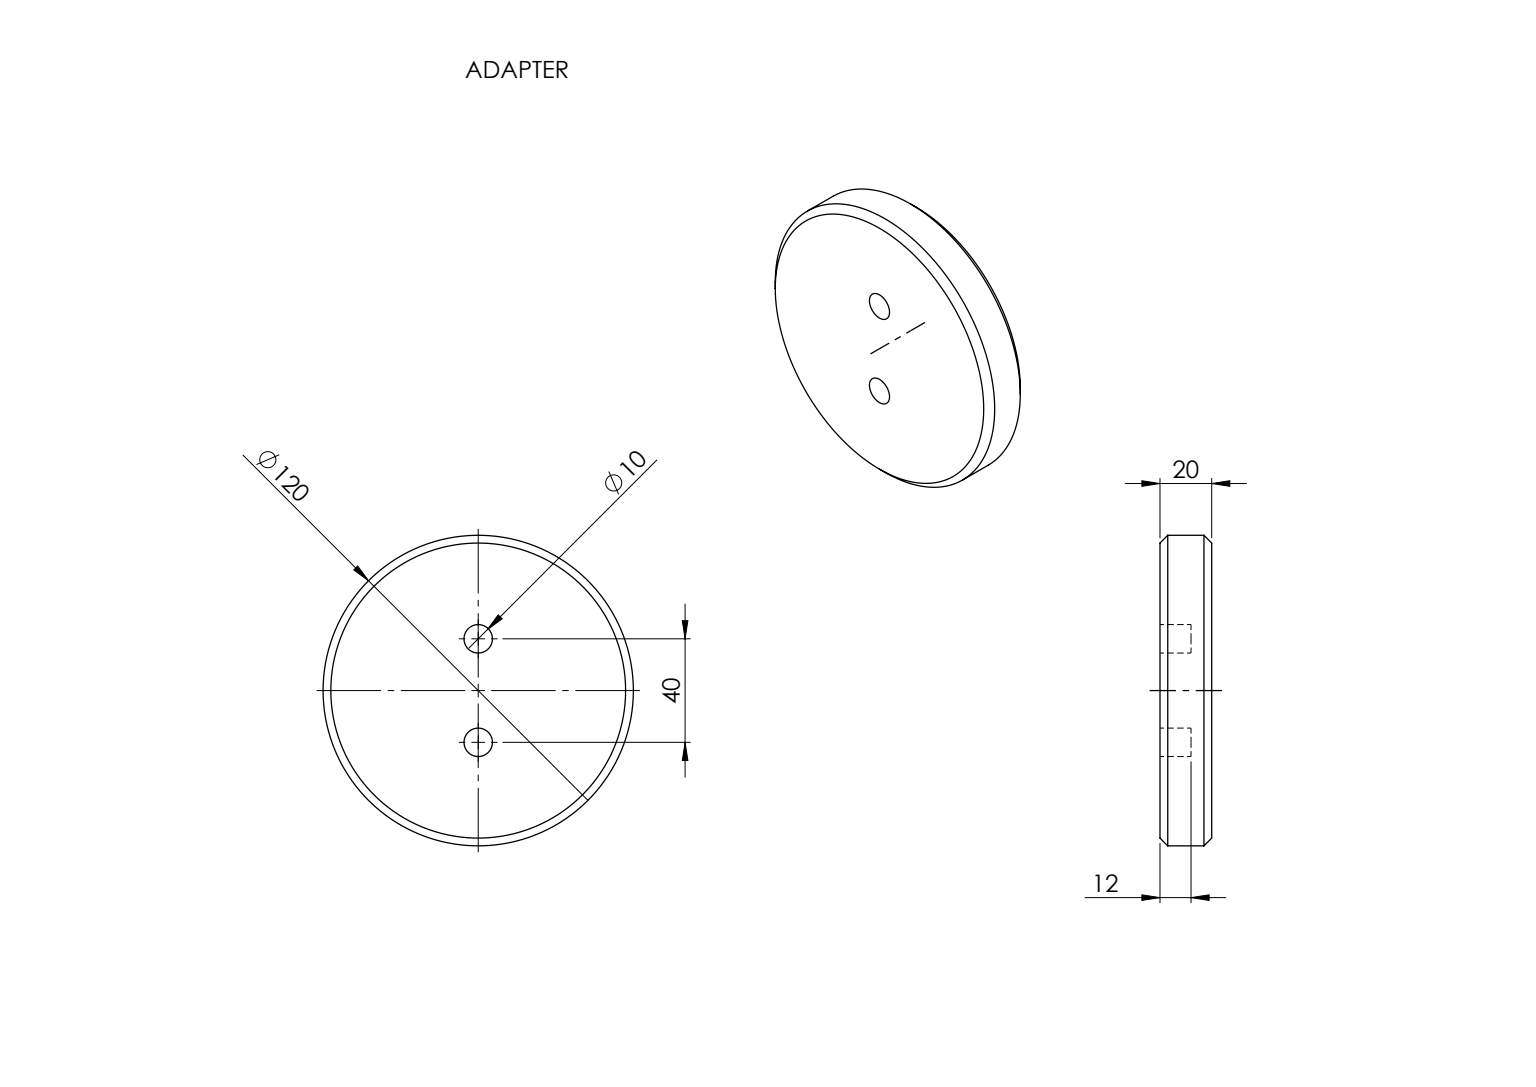
ISO-10303-21;
HEADER;
FILE_DESCRIPTION (('STEP AP203'),
    '1' );
FILE_NAME ('adapter.step',
    '2026-09-28T05:57:06',
    ( '' ),
    ( '' ),
    'SwSTEP 2.0',
    'SolidWorks 2026',
    '' );
FILE_SCHEMA (( 'AUTOMOTIVE_DESIGN' ));
ENDSEC;

DATA;
#193=DIRECTION ( 'NONE',  ( -1.000000000000000000, 0.000000000000000000, 0.000000000000000000 ) ) ;
#236=CARTESIAN_POINT ( 'NONE',  ( 57.00000000000002132, 7.164183775012018789E-15, -220.0000000000000000 ) ) ;
#380=VECTOR ( 'NONE', #39658, 1000.000000000000000 ) ;
#484=ORIENTED_EDGE ( 'NONE', *, *, #2776, .T. ) ;
#740=VERTEX_POINT ( 'NONE', #18224 ) ;
#960=LINE ( 'NONE', #1170, #21072 ) ;
#1101=VECTOR ( 'NONE', #34234, 1000.000000000000114 ) ;
#1161=ORIENTED_EDGE ( 'NONE', *, *, #15645, .F. ) ;
#1170=CARTESIAN_POINT ( 'NONE',  ( -60.00000000000000711, 0.000000000000000000, -223.0000000000000000 ) ) ;
#1309=ORIENTED_EDGE ( 'NONE', *, *, #22453, .T. ) ;
#1322=ORIENTED_EDGE ( 'NONE', *, *, #12215, .F. ) ;
#1370=EDGE_CURVE ( 'NONE', #2118, #27376, #40003, .T. ) ;
#1394=DIRECTION ( 'NONE',  ( -0.000000000000000000, -0.000000000000000000, -1.000000000000000000 ) ) ;
#1563=CIRCLE ( 'NONE', #31918, 57.00000000000002132 ) ;
#1637=VERTEX_POINT ( 'NONE', #18825 ) ;
#1639=CARTESIAN_POINT ( 'NONE',  ( -5.500000000000005329, -20.00000000000000000, -232.0000000000000000 ) ) ;
#1658=APPLICATION_CONTEXT ( 'configuration controlled 3d designs of mechanical parts and assemblies' ) ;
#1713=DIRECTION ( 'NONE',  ( -0.000000000000000000, -0.000000000000000000, -1.000000000000000000 ) ) ;
#1847=CIRCLE ( 'NONE', #5285, 5.500000000000003553 ) ;
#2045=DIRECTION ( 'NONE',  ( -1.000000000000000000, 0.000000000000000000, 0.000000000000000000 ) ) ;
#2118=VERTEX_POINT ( 'NONE', #23558 ) ;
#2181=DIRECTION ( 'NONE',  ( 1.000000000000000000, 0.000000000000000000, 0.000000000000000000 ) ) ;
#2233=CARTESIAN_POINT ( 'NONE',  ( -2.275517850991317657E-15, -20.00000000000000000, -220.0000000000000000 ) ) ;
#2248=CONICAL_SURFACE ( 'NONE', #30493, 57.00000000000002132, 0.7853981633974401744 ) ;
#2458=CARTESIAN_POINT ( 'NONE',  ( -5.500000000000003553, 20.00000000000000000, -220.0000000000000000 ) ) ;
#2487=ORIENTED_EDGE ( 'NONE', *, *, #39307, .F. ) ;
#2493=VERTEX_POINT ( 'NONE', #33169 ) ;
#2732=EDGE_CURVE ( 'NONE', #23382, #12287, #31420, .T. ) ;
#2776=EDGE_CURVE ( 'NONE', #32481, #2118, #24311, .T. ) ;
#2835=DIRECTION ( 'NONE',  ( 0.000000000000000000, 0.000000000000000000, 1.000000000000000000 ) ) ;
#2858=EDGE_CURVE ( 'NONE', #23382, #9326, #21044, .T. ) ;
#3002=ADVANCED_FACE ( 'NONE', ( #15827 ), #29024, .T. ) ;
#3318=CARTESIAN_POINT ( 'NONE',  ( -5.500000000000003553, 20.00000000000000000, -232.0000000000000000 ) ) ;
#3346=CARTESIAN_POINT ( 'NONE',  ( 0.000000000000000000, 20.00000000000000000, -232.0000000000000000 ) ) ;
#3794=PLANE ( 'NONE',  #12718 ) ;
#4148=CARTESIAN_POINT ( 'NONE',  ( 0.000000000000000000, 0.000000000000000000, -220.0000000000000000 ) ) ;
#4242=CONICAL_SURFACE ( 'NONE', #10452, 57.00000000000002132, 0.7853981633974401744 ) ;
#4358=EDGE_CURVE ( 'NONE', #35303, #32901, #36921, .T. ) ;
#4359=DIRECTION ( 'NONE',  ( 0.000000000000000000, 0.000000000000000000, 1.000000000000000000 ) ) ;
#4514=CYLINDRICAL_SURFACE ( 'NONE', #40311, 5.500000000000003553 ) ;
#4553=EDGE_LOOP ( 'NONE', ( #1161, #17163, #11750, #29234 ) ) ;
#5020=DIRECTION ( 'NONE',  ( -0.000000000000000000, -0.000000000000000000, 1.000000000000000000 ) ) ;
#5285=AXIS2_PLACEMENT_3D ( 'NONE', #30798, #38119, #21284 ) ;
#5507=DIRECTION ( 'NONE',  ( 1.000000000000000000, 0.000000000000000000, 0.000000000000000000 ) ) ;
#5518=CONICAL_SURFACE ( 'NONE', #26890, 60.00000000000000711, 0.7853981633974447263 ) ;
#5527=ADVANCED_FACE ( 'NONE', ( #23729 ), #15687, .T. ) ;
#5532=DIRECTION ( 'NONE',  ( 1.000000000000000000, 0.000000000000000000, 0.000000000000000000 ) ) ;
#5685=VERTEX_POINT ( 'NONE', #40743 ) ;
#5789=LINE ( 'NONE', #22397, #7054 ) ;
#6235=DIRECTION ( 'NONE',  ( -0.000000000000000000, -0.000000000000000000, 1.000000000000000000 ) ) ;
#6283=DESIGN_CONTEXT ( 'detailed design', #1658, 'design' ) ;
#6358=AXIS2_PLACEMENT_3D ( 'NONE', #35803, #6235, #193 ) ;
#6631=AXIS2_PLACEMENT_3D ( 'NONE', #37693, #15007, #5532 ) ;
#6876=CIRCLE ( 'NONE', #24103, 5.500000000000003553 ) ;
#6903=CARTESIAN_POINT ( 'NONE',  ( 0.000000000000000000, 0.000000000000000000, -236.9999999999999716 ) ) ;
#7054=VECTOR ( 'NONE', #35785, 1000.000000000000000 ) ;
#7543=FACE_OUTER_BOUND ( 'NONE', #32058, .T. ) ;
#7844=DIRECTION ( 'NONE',  ( -0.000000000000000000, -0.000000000000000000, -1.000000000000000000 ) ) ;
#7898=DIRECTION ( 'NONE',  ( -0.000000000000000000, -0.000000000000000000, 1.000000000000000000 ) ) ;
#8122=DIRECTION ( 'NONE',  ( -0.000000000000000000, -0.000000000000000000, 1.000000000000000000 ) ) ;
#8208=ORIENTED_EDGE ( 'NONE', *, *, #4358, .F. ) ;
#8316=DIRECTION ( 'NONE',  ( 0.000000000000000000, 0.000000000000000000, 1.000000000000000000 ) ) ;
#8492=VERTEX_POINT ( 'NONE', #25338 ) ;
#8866=ORIENTED_EDGE ( 'NONE', *, *, #28211, .T. ) ;
#9072=ORIENTED_EDGE ( 'NONE', *, *, #9834, .F. ) ;
#9326=VERTEX_POINT ( 'NONE', #15542 ) ;
#9491=ORIENTED_EDGE ( 'NONE', *, *, #2858, .T. ) ;
#9834=EDGE_CURVE ( 'NONE', #8492, #5685, #20607, .T. ) ;
#10053=CARTESIAN_POINT ( 'NONE',  ( 60.00000000000000711, 0.000000000000000000, -240.0000000000000000 ) ) ;
#10073=CIRCLE ( 'NONE', #6631, 5.500000000000003553 ) ;
#10213=ORIENTED_EDGE ( 'NONE', *, *, #4358, .T. ) ;
#10322=DIRECTION ( 'NONE',  ( 1.000000000000000000, 0.000000000000000000, 0.000000000000000000 ) ) ;
#10407=ORIENTED_EDGE ( 'NONE', *, *, #16935, .T. ) ;
#10452=AXIS2_PLACEMENT_3D ( 'NONE', #22039, #11663, #35000 ) ;
#10532=ORIENTED_EDGE ( 'NONE', *, *, #33338, .F. ) ;
#10620=EDGE_CURVE ( 'NONE', #5685, #8492, #31701, .T. ) ;
#10627=CARTESIAN_POINT ( 'NONE',  ( 0.000000000000000000, 0.000000000000000000, -223.0000000000000000 ) ) ;
#10691=ORIENTED_EDGE ( 'NONE', *, *, #18172, .T. ) ;
#10913=CYLINDRICAL_SURFACE ( 'NONE', #42182, 5.500000000000003553 ) ;
#10977=DIRECTION ( 'NONE',  ( 1.000000000000000000, 0.000000000000000000, 0.000000000000000000 ) ) ;
#11045=ORIENTED_EDGE ( 'NONE', *, *, #19567, .T. ) ;
#11112=DIRECTION ( 'NONE',  ( 0.000000000000000000, 0.000000000000000000, 1.000000000000000000 ) ) ;
#11162=LINE ( 'NONE', #15034, #36535 ) ;
#11383=ADVANCED_FACE ( 'NONE', ( #21403 ), #24880, .T. ) ;
#11396=DIRECTION ( 'NONE',  ( -1.000000000000000000, 0.000000000000000000, 0.000000000000000000 ) ) ;
#11462=FACE_BOUND ( 'NONE', #29875, .T. ) ;
#11630=ORIENTED_EDGE ( 'NONE', *, *, #12241, .F. ) ;
#11663=DIRECTION ( 'NONE',  ( 0.000000000000000000, 0.000000000000000000, 1.000000000000000000 ) ) ;
#11697=DIRECTION ( 'NONE',  ( 1.000000000000000000, 0.000000000000000000, 0.000000000000000000 ) ) ;
#11750=ORIENTED_EDGE ( 'NONE', *, *, #29145, .T. ) ;
#11756=AXIS2_PLACEMENT_3D ( 'NONE', #2233, #28556, #11697 ) ;
#11785=( GEOMETRIC_REPRESENTATION_CONTEXT ( 3 ) GLOBAL_UNCERTAINTY_ASSIGNED_CONTEXT ( ( #12723 ) ) GLOBAL_UNIT_ASSIGNED_CONTEXT ( ( #35513, #38737, #42168 ) ) REPRESENTATION_CONTEXT ( 'NONE', 'WORKASPACE' ) );
#11914=CARTESIAN_POINT ( 'NONE',  ( -2.275517850991317657E-15, -20.00000000000000000, -232.0000000000000000 ) ) ;
#11964=ORIENTED_EDGE ( 'NONE', *, *, #38901, .F. ) ;
#11965=DIRECTION ( 'NONE',  ( 0.000000000000000000, 0.000000000000000000, -1.000000000000000000 ) ) ;
#12025=DIRECTION ( 'NONE',  ( -0.000000000000000000, -0.000000000000000000, -1.000000000000000000 ) ) ;
#12215=EDGE_CURVE ( 'NONE', #740, #35303, #32992, .T. ) ;
#12241=EDGE_CURVE ( 'NONE', #2493, #27376, #26304, .T. ) ;
#12275=CYLINDRICAL_SURFACE ( 'NONE', #24306, 60.00000000000000711 ) ;
#12287=VERTEX_POINT ( 'NONE', #25670 ) ;
#12718=AXIS2_PLACEMENT_3D ( 'NONE', #21678, #8316, #37442 ) ;
#12723=UNCERTAINTY_MEASURE_WITH_UNIT (LENGTH_MEASURE( 1.000000000000000082E-05 ), #35513, 'distance_accuracy_value', 'NONE');
#12816=SHAPE_REPRESENTATION ( 'adapter', ( #39998 ), #11785 ) ;
#13120=FACE_OUTER_BOUND ( 'NONE', #29690, .T. ) ;
#13284=ADVANCED_FACE ( 'NONE', ( #33374 ), #3794, .T. ) ;
#13467=APPLICATION_CONTEXT ( 'configuration controlled 3d designs of mechanical parts and assemblies' ) ;
#13471=EDGE_LOOP ( 'NONE', ( #17054, #40046, #32542, #32157 ) ) ;
#14188=CARTESIAN_POINT ( 'NONE',  ( 0.000000000000000000, 0.000000000000000000, -223.0000000000000000 ) ) ;
#14397=VERTEX_POINT ( 'NONE', #27211 ) ;
#14563=PRODUCT ( 'adapter', 'adapter', '', ( #16678 ) ) ;
#14656=ORIENTED_EDGE ( 'NONE', *, *, #2732, .F. ) ;
#14767=CARTESIAN_POINT ( 'NONE',  ( 60.00000000000000711, 7.347880794884119933E-15, -223.0000000000000000 ) ) ;
#15007=DIRECTION ( 'NONE',  ( 0.000000000000000000, 0.000000000000000000, 1.000000000000000000 ) ) ;
#15034=CARTESIAN_POINT ( 'NONE',  ( -60.00000000000000711, 7.347880794884119933E-15, -240.0000000000000000 ) ) ;
#15040=CARTESIAN_POINT ( 'NONE',  ( 0.000000000000000000, 0.000000000000000000, -223.0000000000000000 ) ) ;
#15044=AXIS2_PLACEMENT_3D ( 'NONE', #3346, #20365, #23413 ) ;
#15410=CARTESIAN_POINT ( 'NONE',  ( 0.000000000000000000, 0.000000000000000000, -240.0000000000000000 ) ) ;
#15415=SHAPE_REPRESENTATION_RELATIONSHIP ( 'NONE' , 'NONE' ,  #12816, #16028 ) ;
#15542=CARTESIAN_POINT ( 'NONE',  ( 60.00000000000000711, 0.000000000000000000, -223.0000000000000000 ) ) ;
#15645=EDGE_CURVE ( 'NONE', #14397, #5685, #20828, .T. ) ;
#15687=CONICAL_SURFACE ( 'NONE', #28110, 60.00000000000000711, 0.7853981633974447263 ) ;
#15820=DIRECTION ( 'NONE',  ( -0.000000000000000000, -0.000000000000000000, 1.000000000000000000 ) ) ;
#15827=FACE_OUTER_BOUND ( 'NONE', #35717, .T. ) ;
#15849=DIRECTION ( 'NONE',  ( 1.000000000000000000, 0.000000000000000000, -0.000000000000000000 ) ) ;
#15921=PRODUCT_DEFINITION ( 'UNKNOWN', '', #36593, #6283 ) ;
#16028=ADVANCED_BREP_SHAPE_REPRESENTATION ( '', ( #29947, #39998 ), #11785 ) ;
#16120=CARTESIAN_POINT ( 'NONE',  ( -60.00000000000000711, 7.347880794884119933E-15, -223.0000000000000000 ) ) ;
#16275=ADVANCED_FACE ( 'NONE', ( #27640 ), #2248, .T. ) ;
#16443=ORIENTED_EDGE ( 'NONE', *, *, #22506, .F. ) ;
#16678=MECHANICAL_CONTEXT ( 'NONE', #13467, 'mechanical' ) ;
#16734=VERTEX_POINT ( 'NONE', #16120 ) ;
#16893=AXIS2_PLACEMENT_3D ( 'NONE', #25601, #26229, #15849 ) ;
#16935=EDGE_CURVE ( 'NONE', #12287, #23382, #24986, .T. ) ;
#17054=ORIENTED_EDGE ( 'NONE', *, *, #41015, .F. ) ;
#17100=CIRCLE ( 'NONE', #41223, 5.500000000000003553 ) ;
#17163=ORIENTED_EDGE ( 'NONE', *, *, #18172, .F. ) ;
#17263=AXIS2_PLACEMENT_3D ( 'NONE', #39888, #26527, #10322 ) ;
#17268=ORIENTED_EDGE ( 'NONE', *, *, #39307, .T. ) ;
#17292=DIRECTION ( 'NONE',  ( 0.000000000000000000, 0.000000000000000000, -1.000000000000000000 ) ) ;
#17389=AXIS2_PLACEMENT_3D ( 'NONE', #22480, #35023, #35656 ) ;
#17585=AXIS2_PLACEMENT_3D ( 'NONE', #28290, #31537, #2181 ) ;
#18033=CIRCLE ( 'NONE', #29768, 5.500000000000003553 ) ;
#18147=EDGE_CURVE ( 'NONE', #14397, #1637, #1563, .T. ) ;
#18172=EDGE_CURVE ( 'NONE', #1637, #14397, #25684, .T. ) ;
#18224=CARTESIAN_POINT ( 'NONE',  ( 5.500000000000003553, 20.00000000000000000, -232.0000000000000000 ) ) ;
#18549=DIRECTION ( 'NONE',  ( 1.000000000000000000, 0.000000000000000000, 0.000000000000000000 ) ) ;
#18619=ADVANCED_FACE ( 'NONE', ( #41630 ), #12275, .T. ) ;
#18825=CARTESIAN_POINT ( 'NONE',  ( 57.00000000000002132, 0.000000000000000000, -240.0000000000000000 ) ) ;
#19040=ORIENTED_EDGE ( 'NONE', *, *, #41015, .T. ) ;
#19111=PLANE ( 'NONE',  #16893 ) ;
#19567=EDGE_CURVE ( 'NONE', #12287, #16734, #960, .T. ) ;
#19669=ORIENTED_EDGE ( 'NONE', *, *, #25456, .T. ) ;
#19683=VECTOR ( 'NONE', #7898, 1000.000000000000000 ) ;
#20127=ORIENTED_EDGE ( 'NONE', *, *, #18147, .F. ) ;
#20365=DIRECTION ( 'NONE',  ( -0.000000000000000000, -0.000000000000000000, 1.000000000000000000 ) ) ;
#20607=CIRCLE ( 'NONE', #34440, 60.00000000000000711 ) ;
#20828=LINE ( 'NONE', #31208, #36662 ) ;
#20970=FACE_OUTER_BOUND ( 'NONE', #27807, .T. ) ;
#21016=CARTESIAN_POINT ( 'NONE',  ( 0.000000000000000000, 0.000000000000000000, -223.0000000000000000 ) ) ;
#21044=LINE ( 'NONE', #14767, #1101 ) ;
#21072=VECTOR ( 'NONE', #24049, 1000.000000000000114 ) ;
#21276=AXIS2_PLACEMENT_3D ( 'NONE', #29585, #2835, #25721 ) ;
#21284=DIRECTION ( 'NONE',  ( 1.000000000000000000, 0.000000000000000000, 0.000000000000000000 ) ) ;
#21318=EDGE_LOOP ( 'NONE', ( #8208, #41075 ) ) ;
#21403=FACE_OUTER_BOUND ( 'NONE', #13471, .T. ) ;
#21493=CARTESIAN_POINT ( 'NONE',  ( 0.000000000000000000, 20.00000000000000000, -232.0000000000000000 ) ) ;
#21678=CARTESIAN_POINT ( 'NONE',  ( 0.000000000000000000, 20.00000000000000000, -232.0000000000000000 ) ) ;
#21837=DIRECTION ( 'NONE',  ( 1.000000000000000000, 0.000000000000000000, 0.000000000000000000 ) ) ;
#21844=CARTESIAN_POINT ( 'NONE',  ( 0.000000000000000000, 0.000000000000000000, -240.0000000000000000 ) ) ;
#21902=DIRECTION ( 'NONE',  ( 0.000000000000000000, 0.000000000000000000, 1.000000000000000000 ) ) ;
#22039=CARTESIAN_POINT ( 'NONE',  ( 0.000000000000000000, 0.000000000000000000, -240.0000000000000000 ) ) ;
#22127=ORIENTED_EDGE ( 'NONE', *, *, #29145, .F. ) ;
#22183=EDGE_LOOP ( 'NONE', ( #16443, #19669, #8866, #1322 ) ) ;
#22220=CARTESIAN_POINT ( 'NONE',  ( 0.000000000000000000, 0.000000000000000000, -240.0000000000000000 ) ) ;
#22268=CARTESIAN_POINT ( 'NONE',  ( 0.000000000000000000, 0.000000000000000000, -240.0000000000000000 ) ) ;
#22397=CARTESIAN_POINT ( 'NONE',  ( 57.00000000000002132, 0.000000000000000000, -240.0000000000000000 ) ) ;
#22444=EDGE_LOOP ( 'NONE', ( #17268, #41777 ) ) ;
#22453=EDGE_CURVE ( 'NONE', #740, #40819, #10073, .T. ) ;
#22480=CARTESIAN_POINT ( 'NONE',  ( 0.000000000000000000, 0.000000000000000000, -240.0000000000000000 ) ) ;
#22506=EDGE_CURVE ( 'NONE', #40819, #740, #1847, .T. ) ;
#22812=ADVANCED_FACE ( 'NONE', ( #29253 ), #19111, .T. ) ;
#23024=CARTESIAN_POINT ( 'NONE',  ( 0.000000000000000000, 0.000000000000000000, -220.0000000000000000 ) ) ;
#23134=ORIENTED_EDGE ( 'NONE', *, *, #19567, .F. ) ;
#23272=DIRECTION ( 'NONE',  ( -0.000000000000000000, -0.000000000000000000, 1.000000000000000000 ) ) ;
#23382=VERTEX_POINT ( 'NONE', #236 ) ;
#23413=DIRECTION ( 'NONE',  ( 1.000000000000000000, 0.000000000000000000, 0.000000000000000000 ) ) ;
#23558=CARTESIAN_POINT ( 'NONE',  ( -5.500000000000005329, -20.00000000000000000, -220.0000000000000000 ) ) ;
#23563=ORIENTED_EDGE ( 'NONE', *, *, #15645, .T. ) ;
#23591=ADVANCED_FACE ( 'NONE', ( #7543 ), #4514, .F. ) ;
#23644=ORIENTED_EDGE ( 'NONE', *, *, #22453, .F. ) ;
#23729=FACE_OUTER_BOUND ( 'NONE', #36978, .T. ) ;
#23792=FACE_BOUND ( 'NONE', #21318, .T. ) ;
#23829=AXIS2_PLACEMENT_3D ( 'NONE', #23024, #29715, #39831 ) ;
#24049=DIRECTION ( 'NONE',  ( -0.7071067811865451302, 0.000000000000000000, -0.7071067811865500152 ) ) ;
#24103=AXIS2_PLACEMENT_3D ( 'NONE', #11914, #38255, #28773 ) ;
#24229=PLANE ( 'NONE',  #25009 ) ;
#24306=AXIS2_PLACEMENT_3D ( 'NONE', #22220, #31950, #18549 ) ;
#24311=LINE ( 'NONE', #1639, #19683 ) ;
#24322=DIRECTION ( 'NONE',  ( 1.000000000000000000, 0.000000000000000000, 0.000000000000000000 ) ) ;
#24421=CARTESIAN_POINT ( 'NONE',  ( 0.000000000000000000, 0.000000000000000000, -240.0000000000000000 ) ) ;
#24577=DIRECTION ( 'NONE',  ( -1.000000000000000000, 0.000000000000000000, 0.000000000000000000 ) ) ;
#24743=CARTESIAN_POINT ( 'NONE',  ( 0.000000000000000000, 0.000000000000000000, 0.000000000000000000 ) ) ;
#24846=DIRECTION ( 'NONE',  ( 1.000000000000000000, 0.000000000000000000, 0.000000000000000000 ) ) ;
#24880=CYLINDRICAL_SURFACE ( 'NONE', #36889, 60.00000000000000711 ) ;
#24960=PRODUCT_DEFINITION_SHAPE ( 'NONE', 'NONE',  #15921 ) ;
#24986=CIRCLE ( 'NONE', #6358, 57.00000000000002132 ) ;
#25009=AXIS2_PLACEMENT_3D ( 'NONE', #4148, #17292, #27029 ) ;
#25194=EDGE_LOOP ( 'NONE', ( #20127, #23563, #9072, #22127 ) ) ;
#25338=CARTESIAN_POINT ( 'NONE',  ( 60.00000000000000711, 0.000000000000000000, -236.9999999999999716 ) ) ;
#25456=EDGE_CURVE ( 'NONE', #40819, #32901, #42363, .T. ) ;
#25601=CARTESIAN_POINT ( 'NONE',  ( -2.275517850991317657E-15, -20.00000000000000000, -232.0000000000000000 ) ) ;
#25670=CARTESIAN_POINT ( 'NONE',  ( -57.00000000000002132, 0.000000000000000000, -220.0000000000000000 ) ) ;
#25684=CIRCLE ( 'NONE', #17389, 57.00000000000002132 ) ;
#25721=DIRECTION ( 'NONE',  ( 1.000000000000000000, 0.000000000000000000, 0.000000000000000000 ) ) ;
#25731=DIRECTION ( 'NONE',  ( -1.000000000000000000, 0.000000000000000000, 0.000000000000000000 ) ) ;
#25846=ORIENTED_EDGE ( 'NONE', *, *, #1370, .F. ) ;
#25849=VECTOR ( 'NONE', #23272, 1000.000000000000000 ) ;
#26229=DIRECTION ( 'NONE',  ( 0.000000000000000000, 0.000000000000000000, 1.000000000000000000 ) ) ;
#26304=LINE ( 'NONE', #42049, #380 ) ;
#26467=LINE ( 'NONE', #10053, #38727 ) ;
#26527=DIRECTION ( 'NONE',  ( -0.000000000000000000, -0.000000000000000000, 1.000000000000000000 ) ) ;
#26775=ADVANCED_FACE ( 'NONE', ( #28738 ), #4242, .T. ) ;
#26857=AXIS2_PLACEMENT_3D ( 'NONE', #10627, #7844, #27905 ) ;
#26890=AXIS2_PLACEMENT_3D ( 'NONE', #15040, #12025, #24577 ) ;
#26945=ORIENTED_EDGE ( 'NONE', *, *, #27596, .F. ) ;
#26963=DIRECTION ( 'NONE',  ( 0.000000000000000000, 0.000000000000000000, 1.000000000000000000 ) ) ;
#27029=DIRECTION ( 'NONE',  ( -1.000000000000000000, 0.000000000000000000, -0.000000000000000000 ) ) ;
#27059=SHAPE_DEFINITION_REPRESENTATION ( #24960, #12816 ) ;
#27118=FACE_OUTER_BOUND ( 'NONE', #35922, .T. ) ;
#27211=CARTESIAN_POINT ( 'NONE',  ( -57.00000000000002132, 7.164183775012018789E-15, -240.0000000000000000 ) ) ;
#27274=AXIS2_PLACEMENT_3D ( 'NONE', #15410, #11965, #42163 ) ;
#27376=VERTEX_POINT ( 'NONE', #38150 ) ;
#27478=CIRCLE ( 'NONE', #21276, 5.500000000000003553 ) ;
#27596=EDGE_CURVE ( 'NONE', #8492, #9326, #26467, .T. ) ;
#27640=FACE_OUTER_BOUND ( 'NONE', #25194, .T. ) ;
#27750=ORIENTED_EDGE ( 'NONE', *, *, #1370, .T. ) ;
#27805=FACE_OUTER_BOUND ( 'NONE', #31001, .T. ) ;
#27807=EDGE_LOOP ( 'NONE', ( #10407, #32438 ) ) ;
#27905=DIRECTION ( 'NONE',  ( -1.000000000000000000, 0.000000000000000000, 0.000000000000000000 ) ) ;
#28070=CLOSED_SHELL ( 'NONE', ( #32298, #23591, #16275, #39638, #18619, #11383, #3002, #28357, #5527, #26775, #41929, #22812, #29648, #13284 ) ) ;
#28110=AXIS2_PLACEMENT_3D ( 'NONE', #14188, #1713, #11396 ) ;
#28131=ORIENTED_EDGE ( 'NONE', *, *, #12241, .T. ) ;
#28211=EDGE_CURVE ( 'NONE', #32901, #35303, #18033, .T. ) ;
#28287=DIRECTION ( 'NONE',  ( 0.000000000000000000, 0.000000000000000000, 1.000000000000000000 ) ) ;
#28290=CARTESIAN_POINT ( 'NONE',  ( 0.000000000000000000, 20.00000000000000000, -220.0000000000000000 ) ) ;
#28357=ADVANCED_FACE ( 'NONE', ( #23792, #11462, #20970 ), #24229, .F. ) ;
#28372=DIRECTION ( 'NONE',  ( 0.000000000000000000, 0.000000000000000000, 1.000000000000000000 ) ) ;
#28556=DIRECTION ( 'NONE',  ( 0.000000000000000000, 0.000000000000000000, 1.000000000000000000 ) ) ;
#28738=FACE_OUTER_BOUND ( 'NONE', #4553, .T. ) ;
#28773=DIRECTION ( 'NONE',  ( 1.000000000000000000, 0.000000000000000000, 0.000000000000000000 ) ) ;
#29024=PLANE ( 'NONE',  #27274 ) ;
#29145=EDGE_CURVE ( 'NONE', #1637, #8492, #5789, .T. ) ;
#29234=ORIENTED_EDGE ( 'NONE', *, *, #10620, .F. ) ;
#29253=FACE_OUTER_BOUND ( 'NONE', #22444, .T. ) ;
#29585=CARTESIAN_POINT ( 'NONE',  ( -2.275517850991317657E-15, -20.00000000000000000, -220.0000000000000000 ) ) ;
#29648=ADVANCED_FACE ( 'NONE', ( #27118 ), #10913, .F. ) ;
#29690=EDGE_LOOP ( 'NONE', ( #40460, #2487, #28131, #31427 ) ) ;
#29715=DIRECTION ( 'NONE',  ( -0.000000000000000000, -0.000000000000000000, 1.000000000000000000 ) ) ;
#29768=AXIS2_PLACEMENT_3D ( 'NONE', #41737, #21902, #5507 ) ;
#29875=EDGE_LOOP ( 'NONE', ( #34877, #25846 ) ) ;
#29947=MANIFOLD_SOLID_BREP ( 'Cut-Extrude1', #28070 ) ;
#30493=AXIS2_PLACEMENT_3D ( 'NONE', #24421, #28287, #24846 ) ;
#30666=ORIENTED_EDGE ( 'NONE', *, *, #25456, .F. ) ;
#30776=DIRECTION ( 'NONE',  ( -0.7071067811865417996, 8.659560562354863833E-17, 0.7071067811865532349 ) ) ;
#30798=CARTESIAN_POINT ( 'NONE',  ( 0.000000000000000000, 20.00000000000000000, -232.0000000000000000 ) ) ;
#31001=EDGE_LOOP ( 'NONE', ( #14656, #9491, #42149, #23134 ) ) ;
#31125=VECTOR ( 'NONE', #15820, 1000.000000000000000 ) ;
#31208=CARTESIAN_POINT ( 'NONE',  ( -57.00000000000002132, 6.980486755139916067E-15, -240.0000000000000000 ) ) ;
#31420=CIRCLE ( 'NONE', #23829, 57.00000000000002132 ) ;
#31427=ORIENTED_EDGE ( 'NONE', *, *, #34897, .T. ) ;
#31537=DIRECTION ( 'NONE',  ( 0.000000000000000000, 0.000000000000000000, 1.000000000000000000 ) ) ;
#31701=CIRCLE ( 'NONE', #39255, 60.00000000000000711 ) ;
#31918=AXIS2_PLACEMENT_3D ( 'NONE', #21844, #38672, #25731 ) ;
#31950=DIRECTION ( 'NONE',  ( -0.000000000000000000, -0.000000000000000000, 1.000000000000000000 ) ) ;
#32058=EDGE_LOOP ( 'NONE', ( #10532, #484, #27750, #11630 ) ) ;
#32157=ORIENTED_EDGE ( 'NONE', *, *, #38901, .T. ) ;
#32298=ADVANCED_FACE ( 'NONE', ( #40008 ), #36355, .F. ) ;
#32438=ORIENTED_EDGE ( 'NONE', *, *, #2732, .T. ) ;
#32481=VERTEX_POINT ( 'NONE', #40214 ) ;
#32542=ORIENTED_EDGE ( 'NONE', *, *, #27596, .T. ) ;
#32790=CYLINDRICAL_SURFACE ( 'NONE', #17263, 5.500000000000003553 ) ;
#32901=VERTEX_POINT ( 'NONE', #2458 ) ;
#32992=LINE ( 'NONE', #42468, #25849 ) ;
#33169=CARTESIAN_POINT ( 'NONE',  ( 5.500000000000000888, -20.00000000000000000, -232.0000000000000000 ) ) ;
#33232=ORIENTED_EDGE ( 'NONE', *, *, #12215, .T. ) ;
#33338=EDGE_CURVE ( 'NONE', #32481, #2493, #17100, .T. ) ;
#33374=FACE_OUTER_BOUND ( 'NONE', #40398, .T. ) ;
#33463=CARTESIAN_POINT ( 'NONE',  ( -2.275517850991317657E-15, -20.00000000000000000, -232.0000000000000000 ) ) ;
#33874=EDGE_CURVE ( 'NONE', #16734, #9326, #39208, .T. ) ;
#33935=CARTESIAN_POINT ( 'NONE',  ( -2.275517850991317657E-15, -20.00000000000000000, -232.0000000000000000 ) ) ;
#34234=DIRECTION ( 'NONE',  ( 0.7071067811865451302, 8.659560562354904508E-17, -0.7071067811865500152 ) ) ;
#34319=CARTESIAN_POINT ( 'NONE',  ( 5.500000000000003553, 20.00000000000000000, -220.0000000000000000 ) ) ;
#34440=AXIS2_PLACEMENT_3D ( 'NONE', #6903, #26963, #36679 ) ;
#34877=ORIENTED_EDGE ( 'NONE', *, *, #34897, .F. ) ;
#34897=EDGE_CURVE ( 'NONE', #27376, #2118, #27478, .T. ) ;
#35000=DIRECTION ( 'NONE',  ( 1.000000000000000000, 0.000000000000000000, 0.000000000000000000 ) ) ;
#35023=DIRECTION ( 'NONE',  ( 0.000000000000000000, 0.000000000000000000, -1.000000000000000000 ) ) ;
#35303=VERTEX_POINT ( 'NONE', #34319 ) ;
#35488=CARTESIAN_POINT ( 'NONE',  ( 0.000000000000000000, 0.000000000000000000, -236.9999999999999716 ) ) ;
#35513=( LENGTH_UNIT ( ) NAMED_UNIT ( * ) SI_UNIT ( .MILLI., .METRE. ) );
#35656=DIRECTION ( 'NONE',  ( -1.000000000000000000, 0.000000000000000000, 0.000000000000000000 ) ) ;
#35717=EDGE_LOOP ( 'NONE', ( #10691, #38745 ) ) ;
#35785=DIRECTION ( 'NONE',  ( 0.7071067811865417996, 0.000000000000000000, 0.7071067811865532349 ) ) ;
#35803=CARTESIAN_POINT ( 'NONE',  ( 0.000000000000000000, 0.000000000000000000, -220.0000000000000000 ) ) ;
#35922=EDGE_LOOP ( 'NONE', ( #30666, #23644, #33232, #10213 ) ) ;
#36156=ORIENTED_EDGE ( 'NONE', *, *, #22506, .T. ) ;
#36355=CYLINDRICAL_SURFACE ( 'NONE', #15044, 5.500000000000003553 ) ;
#36535=VECTOR ( 'NONE', #37720, 1000.000000000000000 ) ;
#36593=PRODUCT_DEFINITION_FORMATION_WITH_SPECIFIED_SOURCE ( 'ANY', '', #14563, .NOT_KNOWN. ) ;
#36662=VECTOR ( 'NONE', #30776, 1000.000000000000000 ) ;
#36679=DIRECTION ( 'NONE',  ( -1.000000000000000000, 0.000000000000000000, 0.000000000000000000 ) ) ;
#36861=CARTESIAN_POINT ( 'NONE',  ( -5.500000000000003553, 20.00000000000000000, -232.0000000000000000 ) ) ;
#36889=AXIS2_PLACEMENT_3D ( 'NONE', #22268, #5020, #21837 ) ;
#36921=CIRCLE ( 'NONE', #17585, 5.500000000000003553 ) ;
#36978=EDGE_LOOP ( 'NONE', ( #39264, #41213, #11045, #11964 ) ) ;
#37320=DIRECTION ( 'NONE',  ( -0.000000000000000000, -0.000000000000000000, 1.000000000000000000 ) ) ;
#37442=DIRECTION ( 'NONE',  ( 1.000000000000000000, 0.000000000000000000, -0.000000000000000000 ) ) ;
#37550=ORIENTED_EDGE ( 'NONE', *, *, #9834, .T. ) ;
#37641=DIRECTION ( 'NONE',  ( -1.000000000000000000, 0.000000000000000000, 0.000000000000000000 ) ) ;
#37693=CARTESIAN_POINT ( 'NONE',  ( 0.000000000000000000, 20.00000000000000000, -232.0000000000000000 ) ) ;
#37720=DIRECTION ( 'NONE',  ( -0.000000000000000000, -0.000000000000000000, 1.000000000000000000 ) ) ;
#37889=DIRECTION ( 'NONE',  ( 1.000000000000000000, 0.000000000000000000, 0.000000000000000000 ) ) ;
#38119=DIRECTION ( 'NONE',  ( 0.000000000000000000, 0.000000000000000000, 1.000000000000000000 ) ) ;
#38150=CARTESIAN_POINT ( 'NONE',  ( 5.500000000000000888, -20.00000000000000000, -220.0000000000000000 ) ) ;
#38255=DIRECTION ( 'NONE',  ( 0.000000000000000000, 0.000000000000000000, 1.000000000000000000 ) ) ;
#38672=DIRECTION ( 'NONE',  ( 0.000000000000000000, 0.000000000000000000, -1.000000000000000000 ) ) ;
#38727=VECTOR ( 'NONE', #39202, 1000.000000000000000 ) ;
#38737=( NAMED_UNIT ( * ) PLANE_ANGLE_UNIT ( ) SI_UNIT ( $, .RADIAN. ) );
#38745=ORIENTED_EDGE ( 'NONE', *, *, #18147, .T. ) ;
#38901=EDGE_CURVE ( 'NONE', #9326, #16734, #42689, .T. ) ;
#39202=DIRECTION ( 'NONE',  ( -0.000000000000000000, -0.000000000000000000, 1.000000000000000000 ) ) ;
#39208=CIRCLE ( 'NONE', #40569, 60.00000000000000711 ) ;
#39255=AXIS2_PLACEMENT_3D ( 'NONE', #35488, #28372, #2045 ) ;
#39264=ORIENTED_EDGE ( 'NONE', *, *, #2858, .F. ) ;
#39307=EDGE_CURVE ( 'NONE', #2493, #32481, #6876, .T. ) ;
#39638=ADVANCED_FACE ( 'NONE', ( #27805 ), #5518, .T. ) ;
#39658=DIRECTION ( 'NONE',  ( -0.000000000000000000, -0.000000000000000000, 1.000000000000000000 ) ) ;
#39831=DIRECTION ( 'NONE',  ( -1.000000000000000000, 0.000000000000000000, 0.000000000000000000 ) ) ;
#39872=EDGE_LOOP ( 'NONE', ( #37550, #19040, #41433, #26945 ) ) ;
#39888=CARTESIAN_POINT ( 'NONE',  ( -2.275517850991317657E-15, -20.00000000000000000, -232.0000000000000000 ) ) ;
#39998=AXIS2_PLACEMENT_3D ( 'NONE', #24743, #11112, #37889 ) ;
#40003=CIRCLE ( 'NONE', #11756, 5.500000000000003553 ) ;
#40008=FACE_OUTER_BOUND ( 'NONE', #22183, .T. ) ;
#40046=ORIENTED_EDGE ( 'NONE', *, *, #10620, .T. ) ;
#40214=CARTESIAN_POINT ( 'NONE',  ( -5.500000000000005329, -20.00000000000000000, -232.0000000000000000 ) ) ;
#40311=AXIS2_PLACEMENT_3D ( 'NONE', #33463, #37320, #10977 ) ;
#40398=EDGE_LOOP ( 'NONE', ( #1309, #36156 ) ) ;
#40460=ORIENTED_EDGE ( 'NONE', *, *, #2776, .F. ) ;
#40569=AXIS2_PLACEMENT_3D ( 'NONE', #21016, #1394, #37641 ) ;
#40587=DIRECTION ( 'NONE',  ( 1.000000000000000000, 0.000000000000000000, 0.000000000000000000 ) ) ;
#40743=CARTESIAN_POINT ( 'NONE',  ( -60.00000000000000711, 7.347880794884119933E-15, -236.9999999999999716 ) ) ;
#40819=VERTEX_POINT ( 'NONE', #36861 ) ;
#41015=EDGE_CURVE ( 'NONE', #5685, #16734, #11162, .T. ) ;
#41075=ORIENTED_EDGE ( 'NONE', *, *, #28211, .F. ) ;
#41213=ORIENTED_EDGE ( 'NONE', *, *, #16935, .F. ) ;
#41223=AXIS2_PLACEMENT_3D ( 'NONE', #33935, #4359, #40587 ) ;
#41433=ORIENTED_EDGE ( 'NONE', *, *, #33874, .T. ) ;
#41630=FACE_OUTER_BOUND ( 'NONE', #39872, .T. ) ;
#41737=CARTESIAN_POINT ( 'NONE',  ( 0.000000000000000000, 20.00000000000000000, -220.0000000000000000 ) ) ;
#41777=ORIENTED_EDGE ( 'NONE', *, *, #33338, .T. ) ;
#41929=ADVANCED_FACE ( 'NONE', ( #13120 ), #32790, .F. ) ;
#42049=CARTESIAN_POINT ( 'NONE',  ( 5.500000000000000888, -20.00000000000000000, -232.0000000000000000 ) ) ;
#42149=ORIENTED_EDGE ( 'NONE', *, *, #33874, .F. ) ;
#42163=DIRECTION ( 'NONE',  ( -1.000000000000000000, 0.000000000000000000, -0.000000000000000000 ) ) ;
#42168=( NAMED_UNIT ( * ) SI_UNIT ( $, .STERADIAN. ) SOLID_ANGLE_UNIT ( ) );
#42182=AXIS2_PLACEMENT_3D ( 'NONE', #21493, #8122, #24322 ) ;
#42363=LINE ( 'NONE', #3318, #31125 ) ;
#42468=CARTESIAN_POINT ( 'NONE',  ( 5.500000000000003553, 20.00000000000000000, -232.0000000000000000 ) ) ;
#42689=CIRCLE ( 'NONE', #26857, 60.00000000000000711 ) ;
#42725=COLOUR_RGB('Light Gray', 0.72549020, 0.75294118, 0.79215686);
#42726=FILL_AREA_STYLE_COLOUR('',#42725);
#42727=FILL_AREA_STYLE('',(#42726));
#42728=SURFACE_STYLE_FILL_AREA(#42727);
#42729=SURFACE_SIDE_STYLE('',(#42728));
#42730=SURFACE_STYLE_USAGE(.BOTH.,#42729);
#42731=PRESENTATION_STYLE_ASSIGNMENT((#42730));
#42739=STYLED_ITEM('',(#42731),#29947);
#42740=MECHANICAL_DESIGN_GEOMETRIC_PRESENTATION_REPRESENTATION('',(#42739),#11785);
ENDSEC;
END-ISO-10303-21;
